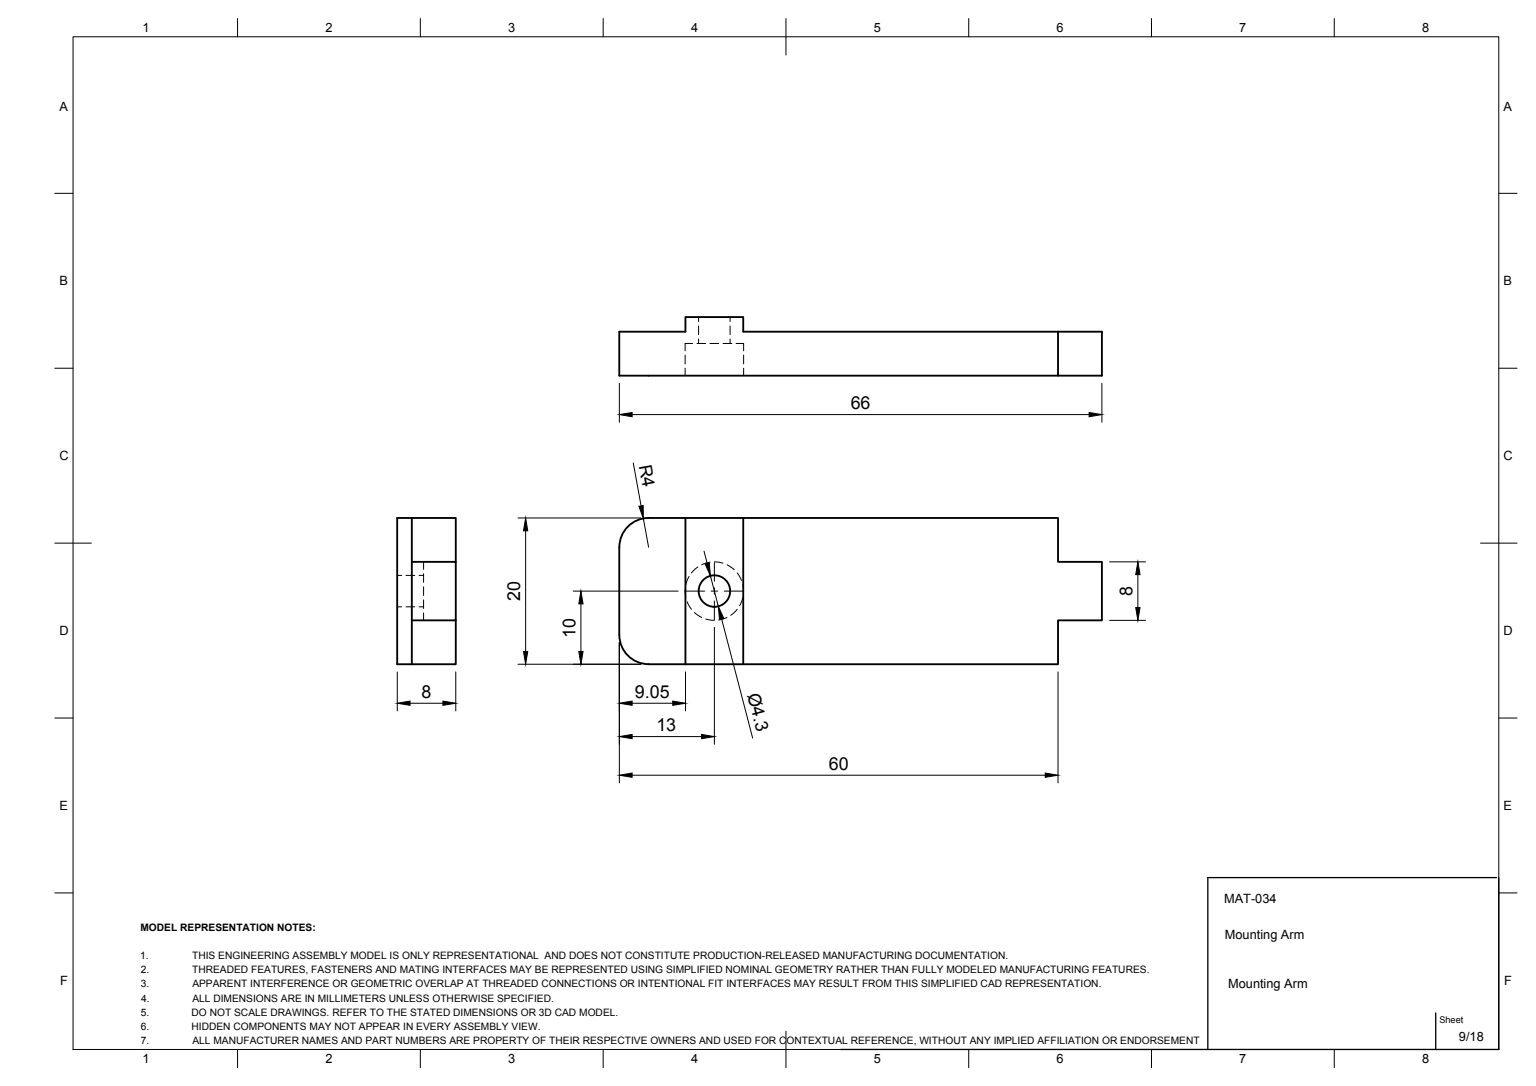
ISO-10303-21;
HEADER;
/* Generated by software containing ST-Developer
 * from STEP Tools, Inc. (www.steptools.com) 
 */

FILE_DESCRIPTION(
/* description */ ('STEP AP214'),
/* implementation_level */ '2;1');

FILE_NAME(
/* name */ 'Mounting Arm.step',
/* time_stamp */ '2026-11-14T09:24:36-08:00',
/* author */ (''),
/* organization */ (''),
/* preprocessor_version */ 'ST-DEVELOPER v20.2',
/* originating_system */ 'Autodesk Translation Framework v15.17.0.0',
/* authorisation */ '');

FILE_SCHEMA (('AUTOMOTIVE_DESIGN { 1 0 10303 214 3 1 1 }'));
ENDSEC;

DATA;
#10=MECHANICAL_DESIGN_GEOMETRIC_PRESENTATION_REPRESENTATION('',(#215),#18867);
#183=SHAPE_REPRESENTATION_RELATIONSHIP('SRR','None',#18947,#199);
#199=ADVANCED_BREP_SHAPE_REPRESENTATION('',(#239),#18863);
#215=STYLED_ITEM('',(#19026),#239);
#239=MANIFOLD_SOLID_BREP('Body1',#10970);
#362=FACE_BOUND('',#1945,.T.);
#363=FACE_BOUND('',#1952,.T.);
#364=FACE_BOUND('',#1956,.T.);
#686=PLANE('',#12091);
#687=PLANE('',#12094);
#688=PLANE('',#12095);
#689=PLANE('',#12096);
#690=PLANE('',#12097);
#691=PLANE('',#12098);
#692=PLANE('',#12099);
#693=PLANE('',#12100);
#694=PLANE('',#12103);
#695=PLANE('',#12104);
#696=PLANE('',#12105);
#697=PLANE('',#12106);
#698=PLANE('',#12107);
#699=PLANE('',#12108);
#700=PLANE('',#12111);
#1228=FACE_OUTER_BOUND('',#1935,.T.);
#1229=FACE_OUTER_BOUND('',#1936,.T.);
#1230=FACE_OUTER_BOUND('',#1937,.T.);
#1231=FACE_OUTER_BOUND('',#1938,.T.);
#1232=FACE_OUTER_BOUND('',#1939,.T.);
#1233=FACE_OUTER_BOUND('',#1940,.T.);
#1234=FACE_OUTER_BOUND('',#1941,.T.);
#1235=FACE_OUTER_BOUND('',#1942,.T.);
#1236=FACE_OUTER_BOUND('',#1943,.T.);
#1237=FACE_OUTER_BOUND('',#1944,.T.);
#1238=FACE_OUTER_BOUND('',#1946,.T.);
#1239=FACE_OUTER_BOUND('',#1947,.T.);
#1240=FACE_OUTER_BOUND('',#1948,.T.);
#1241=FACE_OUTER_BOUND('',#1949,.T.);
#1242=FACE_OUTER_BOUND('',#1950,.T.);
#1243=FACE_OUTER_BOUND('',#1951,.T.);
#1244=FACE_OUTER_BOUND('',#1953,.T.);
#1245=FACE_OUTER_BOUND('',#1954,.T.);
#1246=FACE_OUTER_BOUND('',#1955,.T.);
#1935=EDGE_LOOP('',(#9768,#9769,#9770,#9771));
#1936=EDGE_LOOP('',(#9772,#9773,#9774,#9775));
#1937=EDGE_LOOP('',(#9776,#9777,#9778,#9779,#9780,#9781));
#1938=EDGE_LOOP('',(#9782,#9783,#9784,#9785,#9786,#9787,#9788,#9789));
#1939=EDGE_LOOP('',(#9790,#9791,#9792,#9793));
#1940=EDGE_LOOP('',(#9794,#9795,#9796,#9797));
#1941=EDGE_LOOP('',(#9798,#9799,#9800,#9801,#9802,#9803,#9804,#9805));
#1942=EDGE_LOOP('',(#9806,#9807,#9808,#9809,#9810,#9811,#9812,#9813));
#1943=EDGE_LOOP('',(#9814,#9815,#9816,#9817));
#1944=EDGE_LOOP('',(#9818,#9819,#9820,#9821,#9822,#9823,#9824,#9825,#9826,
#9827));
#1945=EDGE_LOOP('',(#9828));
#1946=EDGE_LOOP('',(#9829,#9830,#9831,#9832));
#1947=EDGE_LOOP('',(#9833,#9834,#9835,#9836));
#1948=EDGE_LOOP('',(#9837,#9838,#9839,#9840));
#1949=EDGE_LOOP('',(#9841,#9842,#9843,#9844));
#1950=EDGE_LOOP('',(#9845,#9846,#9847,#9848));
#1951=EDGE_LOOP('',(#9849,#9850,#9851,#9852));
#1952=EDGE_LOOP('',(#9853));
#1953=EDGE_LOOP('',(#9854,#9855,#9856,#9857));
#1954=EDGE_LOOP('',(#9858,#9859,#9860,#9861));
#1955=EDGE_LOOP('',(#9862));
#1956=EDGE_LOOP('',(#9863));
#2964=LINE('',#18390,#3978);
#2965=LINE('',#18396,#3979);
#2966=LINE('',#18401,#3980);
#2967=LINE('',#18405,#3981);
#2968=LINE('',#18409,#3982);
#2969=LINE('',#18410,#3983);
#2970=LINE('',#18414,#3984);
#2971=LINE('',#18416,#3985);
#2972=LINE('',#18418,#3986);
#2973=LINE('',#18420,#3987);
#2974=LINE('',#18422,#3988);
#2975=LINE('',#18424,#3989);
#2976=LINE('',#18426,#3990);
#2977=LINE('',#18427,#3991);
#2978=LINE('',#18430,#3992);
#2979=LINE('',#18432,#3993);
#2980=LINE('',#18433,#3994);
#2981=LINE('',#18436,#3995);
#2982=LINE('',#18438,#3996);
#2983=LINE('',#18439,#3997);
#2984=LINE('',#18442,#3998);
#2985=LINE('',#18443,#3999);
#2986=LINE('',#18445,#4000);
#2987=LINE('',#18447,#4001);
#2988=LINE('',#18448,#4002);
#2989=LINE('',#18451,#4003);
#2990=LINE('',#18452,#4004);
#2991=LINE('',#18454,#4005);
#2992=LINE('',#18456,#4006);
#2993=LINE('',#18457,#4007);
#2994=LINE('',#18460,#4008);
#2995=LINE('',#18462,#4009);
#2996=LINE('',#18463,#4010);
#2997=LINE('',#18467,#4011);
#2998=LINE('',#18469,#4012);
#2999=LINE('',#18470,#4013);
#3000=LINE('',#18473,#4014);
#3001=LINE('',#18475,#4015);
#3002=LINE('',#18478,#4016);
#3003=LINE('',#18480,#4017);
#3978=VECTOR('',#15076,3.99999999999999);
#3979=VECTOR('',#15083,2.15);
#3980=VECTOR('',#15088,1000.);
#3981=VECTOR('',#15091,1000.);
#3982=VECTOR('',#15094,1000.);
#3983=VECTOR('',#15095,1000.);
#3984=VECTOR('',#15098,1000.);
#3985=VECTOR('',#15099,1000.);
#3986=VECTOR('',#15100,1000.);
#3987=VECTOR('',#15101,1000.);
#3988=VECTOR('',#15102,1000.);
#3989=VECTOR('',#15103,1000.);
#3990=VECTOR('',#15104,1000.);
#3991=VECTOR('',#15105,1000.);
#3992=VECTOR('',#15108,1000.);
#3993=VECTOR('',#15109,1000.);
#3994=VECTOR('',#15110,1000.);
#3995=VECTOR('',#15113,1000.);
#3996=VECTOR('',#15114,1000.);
#3997=VECTOR('',#15115,1000.);
#3998=VECTOR('',#15118,1000.);
#3999=VECTOR('',#15119,1000.);
#4000=VECTOR('',#15120,1000.);
#4001=VECTOR('',#15121,1000.);
#4002=VECTOR('',#15122,1000.);
#4003=VECTOR('',#15125,1000.);
#4004=VECTOR('',#15126,1000.);
#4005=VECTOR('',#15127,1000.);
#4006=VECTOR('',#15128,1000.);
#4007=VECTOR('',#15129,1000.);
#4008=VECTOR('',#15132,1000.);
#4009=VECTOR('',#15133,1000.);
#4010=VECTOR('',#15134,1000.);
#4011=VECTOR('',#15139,1000.);
#4012=VECTOR('',#15140,1000.);
#4013=VECTOR('',#15141,1000.);
#4014=VECTOR('',#15146,1000.);
#4015=VECTOR('',#15149,1000.);
#4016=VECTOR('',#15154,1000.);
#4017=VECTOR('',#15157,1000.);
#4480=CIRCLE('',#12086,4.);
#4481=CIRCLE('',#12087,3.99999999999999);
#4482=CIRCLE('',#12089,2.15);
#4483=CIRCLE('',#12090,2.15);
#4484=CIRCLE('',#12092,4.);
#4485=CIRCLE('',#12093,4.);
#4486=CIRCLE('',#12101,4.);
#4487=CIRCLE('',#12102,4.);
#5456=VERTEX_POINT('',#18387);
#5457=VERTEX_POINT('',#18389);
#5458=VERTEX_POINT('',#18393);
#5459=VERTEX_POINT('',#18395);
#5460=VERTEX_POINT('',#18399);
#5461=VERTEX_POINT('',#18400);
#5462=VERTEX_POINT('',#18402);
#5463=VERTEX_POINT('',#18404);
#5464=VERTEX_POINT('',#18406);
#5465=VERTEX_POINT('',#18408);
#5466=VERTEX_POINT('',#18412);
#5467=VERTEX_POINT('',#18413);
#5468=VERTEX_POINT('',#18415);
#5469=VERTEX_POINT('',#18417);
#5470=VERTEX_POINT('',#18419);
#5471=VERTEX_POINT('',#18421);
#5472=VERTEX_POINT('',#18423);
#5473=VERTEX_POINT('',#18425);
#5474=VERTEX_POINT('',#18429);
#5475=VERTEX_POINT('',#18431);
#5476=VERTEX_POINT('',#18435);
#5477=VERTEX_POINT('',#18437);
#5478=VERTEX_POINT('',#18441);
#5479=VERTEX_POINT('',#18444);
#5480=VERTEX_POINT('',#18446);
#5481=VERTEX_POINT('',#18450);
#5482=VERTEX_POINT('',#18453);
#5483=VERTEX_POINT('',#18455);
#5484=VERTEX_POINT('',#18459);
#5485=VERTEX_POINT('',#18461);
#5486=VERTEX_POINT('',#18466);
#5487=VERTEX_POINT('',#18468);
#6917=EDGE_CURVE('',#5456,#5456,#4480,.T.);
#6918=EDGE_CURVE('',#5456,#5457,#2964,.T.);
#6919=EDGE_CURVE('',#5457,#5457,#4481,.T.);
#6920=EDGE_CURVE('',#5458,#5458,#4482,.T.);
#6921=EDGE_CURVE('',#5458,#5459,#2965,.T.);
#6922=EDGE_CURVE('',#5459,#5459,#4483,.T.);
#6923=EDGE_CURVE('',#5460,#5461,#2966,.T.);
#6924=EDGE_CURVE('',#5460,#5462,#4484,.T.);
#6925=EDGE_CURVE('',#5463,#5462,#2967,.T.);
#6926=EDGE_CURVE('',#5463,#5464,#4485,.T.);
#6927=EDGE_CURVE('',#5465,#5464,#2968,.T.);
#6928=EDGE_CURVE('',#5461,#5465,#2969,.T.);
#6929=EDGE_CURVE('',#5466,#5467,#2970,.T.);
#6930=EDGE_CURVE('',#5468,#5466,#2971,.T.);
#6931=EDGE_CURVE('',#5469,#5468,#2972,.T.);
#6932=EDGE_CURVE('',#5470,#5469,#2973,.T.);
#6933=EDGE_CURVE('',#5471,#5470,#2974,.T.);
#6934=EDGE_CURVE('',#5471,#5472,#2975,.T.);
#6935=EDGE_CURVE('',#5473,#5472,#2976,.T.);
#6936=EDGE_CURVE('',#5467,#5473,#2977,.T.);
#6937=EDGE_CURVE('',#5474,#5472,#2978,.T.);
#6938=EDGE_CURVE('',#5475,#5474,#2979,.T.);
#6939=EDGE_CURVE('',#5475,#5473,#2980,.T.);
#6940=EDGE_CURVE('',#5469,#5476,#2981,.T.);
#6941=EDGE_CURVE('',#5477,#5468,#2982,.T.);
#6942=EDGE_CURVE('',#5476,#5477,#2983,.T.);
#6943=EDGE_CURVE('',#5478,#5475,#2984,.T.);
#6944=EDGE_CURVE('',#5478,#5460,#2985,.T.);
#6945=EDGE_CURVE('',#5479,#5461,#2986,.T.);
#6946=EDGE_CURVE('',#5480,#5479,#2987,.T.);
#6947=EDGE_CURVE('',#5480,#5467,#2988,.T.);
#6948=EDGE_CURVE('',#5464,#5481,#2989,.T.);
#6949=EDGE_CURVE('',#5477,#5481,#2990,.T.);
#6950=EDGE_CURVE('',#5482,#5466,#2991,.T.);
#6951=EDGE_CURVE('',#5483,#5482,#2992,.T.);
#6952=EDGE_CURVE('',#5483,#5465,#2993,.T.);
#6953=EDGE_CURVE('',#5462,#5484,#2994,.T.);
#6954=EDGE_CURVE('',#5485,#5484,#2995,.T.);
#6955=EDGE_CURVE('',#5485,#5463,#2996,.T.);
#6956=EDGE_CURVE('',#5484,#5478,#4486,.T.);
#6957=EDGE_CURVE('',#5486,#5474,#2997,.T.);
#6958=EDGE_CURVE('',#5487,#5486,#2998,.T.);
#6959=EDGE_CURVE('',#5487,#5476,#2999,.T.);
#6960=EDGE_CURVE('',#5481,#5485,#4487,.T.);
#6961=EDGE_CURVE('',#5486,#5471,#3000,.T.);
#6962=EDGE_CURVE('',#5470,#5487,#3001,.T.);
#6963=EDGE_CURVE('',#5482,#5480,#3002,.T.);
#6964=EDGE_CURVE('',#5479,#5483,#3003,.T.);
#9768=ORIENTED_EDGE('',*,*,#6917,.F.);
#9769=ORIENTED_EDGE('',*,*,#6918,.T.);
#9770=ORIENTED_EDGE('',*,*,#6919,.T.);
#9771=ORIENTED_EDGE('',*,*,#6918,.F.);
#9772=ORIENTED_EDGE('',*,*,#6920,.F.);
#9773=ORIENTED_EDGE('',*,*,#6921,.T.);
#9774=ORIENTED_EDGE('',*,*,#6922,.T.);
#9775=ORIENTED_EDGE('',*,*,#6921,.F.);
#9776=ORIENTED_EDGE('',*,*,#6923,.F.);
#9777=ORIENTED_EDGE('',*,*,#6924,.T.);
#9778=ORIENTED_EDGE('',*,*,#6925,.F.);
#9779=ORIENTED_EDGE('',*,*,#6926,.T.);
#9780=ORIENTED_EDGE('',*,*,#6927,.F.);
#9781=ORIENTED_EDGE('',*,*,#6928,.F.);
#9782=ORIENTED_EDGE('',*,*,#6929,.F.);
#9783=ORIENTED_EDGE('',*,*,#6930,.F.);
#9784=ORIENTED_EDGE('',*,*,#6931,.F.);
#9785=ORIENTED_EDGE('',*,*,#6932,.F.);
#9786=ORIENTED_EDGE('',*,*,#6933,.F.);
#9787=ORIENTED_EDGE('',*,*,#6934,.T.);
#9788=ORIENTED_EDGE('',*,*,#6935,.F.);
#9789=ORIENTED_EDGE('',*,*,#6936,.F.);
#9790=ORIENTED_EDGE('',*,*,#6937,.F.);
#9791=ORIENTED_EDGE('',*,*,#6938,.F.);
#9792=ORIENTED_EDGE('',*,*,#6939,.T.);
#9793=ORIENTED_EDGE('',*,*,#6935,.T.);
#9794=ORIENTED_EDGE('',*,*,#6940,.F.);
#9795=ORIENTED_EDGE('',*,*,#6931,.T.);
#9796=ORIENTED_EDGE('',*,*,#6941,.F.);
#9797=ORIENTED_EDGE('',*,*,#6942,.F.);
#9798=ORIENTED_EDGE('',*,*,#6943,.F.);
#9799=ORIENTED_EDGE('',*,*,#6944,.T.);
#9800=ORIENTED_EDGE('',*,*,#6923,.T.);
#9801=ORIENTED_EDGE('',*,*,#6945,.F.);
#9802=ORIENTED_EDGE('',*,*,#6946,.F.);
#9803=ORIENTED_EDGE('',*,*,#6947,.T.);
#9804=ORIENTED_EDGE('',*,*,#6936,.T.);
#9805=ORIENTED_EDGE('',*,*,#6939,.F.);
#9806=ORIENTED_EDGE('',*,*,#6927,.T.);
#9807=ORIENTED_EDGE('',*,*,#6948,.T.);
#9808=ORIENTED_EDGE('',*,*,#6949,.F.);
#9809=ORIENTED_EDGE('',*,*,#6941,.T.);
#9810=ORIENTED_EDGE('',*,*,#6930,.T.);
#9811=ORIENTED_EDGE('',*,*,#6950,.F.);
#9812=ORIENTED_EDGE('',*,*,#6951,.F.);
#9813=ORIENTED_EDGE('',*,*,#6952,.T.);
#9814=ORIENTED_EDGE('',*,*,#6925,.T.);
#9815=ORIENTED_EDGE('',*,*,#6953,.T.);
#9816=ORIENTED_EDGE('',*,*,#6954,.F.);
#9817=ORIENTED_EDGE('',*,*,#6955,.T.);
#9818=ORIENTED_EDGE('',*,*,#6954,.T.);
#9819=ORIENTED_EDGE('',*,*,#6956,.T.);
#9820=ORIENTED_EDGE('',*,*,#6943,.T.);
#9821=ORIENTED_EDGE('',*,*,#6938,.T.);
#9822=ORIENTED_EDGE('',*,*,#6957,.F.);
#9823=ORIENTED_EDGE('',*,*,#6958,.F.);
#9824=ORIENTED_EDGE('',*,*,#6959,.T.);
#9825=ORIENTED_EDGE('',*,*,#6942,.T.);
#9826=ORIENTED_EDGE('',*,*,#6949,.T.);
#9827=ORIENTED_EDGE('',*,*,#6960,.T.);
#9828=ORIENTED_EDGE('',*,*,#6919,.F.);
#9829=ORIENTED_EDGE('',*,*,#6937,.T.);
#9830=ORIENTED_EDGE('',*,*,#6934,.F.);
#9831=ORIENTED_EDGE('',*,*,#6961,.F.);
#9832=ORIENTED_EDGE('',*,*,#6957,.T.);
#9833=ORIENTED_EDGE('',*,*,#6940,.T.);
#9834=ORIENTED_EDGE('',*,*,#6959,.F.);
#9835=ORIENTED_EDGE('',*,*,#6962,.F.);
#9836=ORIENTED_EDGE('',*,*,#6932,.T.);
#9837=ORIENTED_EDGE('',*,*,#6961,.T.);
#9838=ORIENTED_EDGE('',*,*,#6933,.T.);
#9839=ORIENTED_EDGE('',*,*,#6962,.T.);
#9840=ORIENTED_EDGE('',*,*,#6958,.T.);
#9841=ORIENTED_EDGE('',*,*,#6929,.T.);
#9842=ORIENTED_EDGE('',*,*,#6947,.F.);
#9843=ORIENTED_EDGE('',*,*,#6963,.F.);
#9844=ORIENTED_EDGE('',*,*,#6950,.T.);
#9845=ORIENTED_EDGE('',*,*,#6928,.T.);
#9846=ORIENTED_EDGE('',*,*,#6952,.F.);
#9847=ORIENTED_EDGE('',*,*,#6964,.F.);
#9848=ORIENTED_EDGE('',*,*,#6945,.T.);
#9849=ORIENTED_EDGE('',*,*,#6951,.T.);
#9850=ORIENTED_EDGE('',*,*,#6963,.T.);
#9851=ORIENTED_EDGE('',*,*,#6946,.T.);
#9852=ORIENTED_EDGE('',*,*,#6964,.T.);
#9853=ORIENTED_EDGE('',*,*,#6920,.T.);
#9854=ORIENTED_EDGE('',*,*,#6956,.F.);
#9855=ORIENTED_EDGE('',*,*,#6953,.F.);
#9856=ORIENTED_EDGE('',*,*,#6924,.F.);
#9857=ORIENTED_EDGE('',*,*,#6944,.F.);
#9858=ORIENTED_EDGE('',*,*,#6960,.F.);
#9859=ORIENTED_EDGE('',*,*,#6948,.F.);
#9860=ORIENTED_EDGE('',*,*,#6926,.F.);
#9861=ORIENTED_EDGE('',*,*,#6955,.F.);
#9862=ORIENTED_EDGE('',*,*,#6917,.T.);
#9863=ORIENTED_EDGE('',*,*,#6922,.F.);
#10337=CYLINDRICAL_SURFACE('',#12085,3.99999999999999);
#10338=CYLINDRICAL_SURFACE('',#12088,2.15);
#10339=CYLINDRICAL_SURFACE('',#12109,4.);
#10340=CYLINDRICAL_SURFACE('',#12110,4.);
#10865=ADVANCED_FACE('',(#1228),#10337,.F.);
#10866=ADVANCED_FACE('',(#1229),#10338,.F.);
#10867=ADVANCED_FACE('',(#1230),#686,.F.);
#10868=ADVANCED_FACE('',(#1231),#687,.F.);
#10869=ADVANCED_FACE('',(#1232),#688,.F.);
#10870=ADVANCED_FACE('',(#1233),#689,.F.);
#10871=ADVANCED_FACE('',(#1234),#690,.F.);
#10872=ADVANCED_FACE('',(#1235),#691,.F.);
#10873=ADVANCED_FACE('',(#1236),#692,.F.);
#10874=ADVANCED_FACE('',(#1237,#362),#693,.T.);
#10875=ADVANCED_FACE('',(#1238),#694,.F.);
#10876=ADVANCED_FACE('',(#1239),#695,.F.);
#10877=ADVANCED_FACE('',(#1240),#696,.T.);
#10878=ADVANCED_FACE('',(#1241),#697,.F.);
#10879=ADVANCED_FACE('',(#1242),#698,.F.);
#10880=ADVANCED_FACE('',(#1243,#363),#699,.T.);
#10881=ADVANCED_FACE('',(#1244),#10339,.T.);
#10882=ADVANCED_FACE('',(#1245),#10340,.T.);
#10883=ADVANCED_FACE('',(#1246,#364),#700,.F.);
#10970=CLOSED_SHELL('',(#10865,#10866,#10867,#10868,#10869,#10870,#10871,
#10872,#10873,#10874,#10875,#10876,#10877,#10878,#10879,#10880,#10881,#10882,
#10883));
#12084=AXIS2_PLACEMENT_3D('',#18385,#15070,#15071);
#12085=AXIS2_PLACEMENT_3D('',#18386,#15072,#15073);
#12086=AXIS2_PLACEMENT_3D('',#18388,#15074,#15075);
#12087=AXIS2_PLACEMENT_3D('',#18391,#15077,#15078);
#12088=AXIS2_PLACEMENT_3D('',#18392,#15079,#15080);
#12089=AXIS2_PLACEMENT_3D('',#18394,#15081,#15082);
#12090=AXIS2_PLACEMENT_3D('',#18397,#15084,#15085);
#12091=AXIS2_PLACEMENT_3D('',#18398,#15086,#15087);
#12092=AXIS2_PLACEMENT_3D('',#18403,#15089,#15090);
#12093=AXIS2_PLACEMENT_3D('',#18407,#15092,#15093);
#12094=AXIS2_PLACEMENT_3D('',#18411,#15096,#15097);
#12095=AXIS2_PLACEMENT_3D('',#18428,#15106,#15107);
#12096=AXIS2_PLACEMENT_3D('',#18434,#15111,#15112);
#12097=AXIS2_PLACEMENT_3D('',#18440,#15116,#15117);
#12098=AXIS2_PLACEMENT_3D('',#18449,#15123,#15124);
#12099=AXIS2_PLACEMENT_3D('',#18458,#15130,#15131);
#12100=AXIS2_PLACEMENT_3D('',#18464,#15135,#15136);
#12101=AXIS2_PLACEMENT_3D('',#18465,#15137,#15138);
#12102=AXIS2_PLACEMENT_3D('',#18471,#15142,#15143);
#12103=AXIS2_PLACEMENT_3D('',#18472,#15144,#15145);
#12104=AXIS2_PLACEMENT_3D('',#18474,#15147,#15148);
#12105=AXIS2_PLACEMENT_3D('',#18476,#15150,#15151);
#12106=AXIS2_PLACEMENT_3D('',#18477,#15152,#15153);
#12107=AXIS2_PLACEMENT_3D('',#18479,#15155,#15156);
#12108=AXIS2_PLACEMENT_3D('',#18481,#15158,#15159);
#12109=AXIS2_PLACEMENT_3D('',#18482,#15160,#15161);
#12110=AXIS2_PLACEMENT_3D('',#18483,#15162,#15163);
#12111=AXIS2_PLACEMENT_3D('',#18484,#15164,#15165);
#15070=DIRECTION('axis',(0.,0.,1.));
#15071=DIRECTION('refdir',(1.,0.,0.));
#15072=DIRECTION('center_axis',(0.,0.,1.));
#15073=DIRECTION('ref_axis',(1.,0.,0.));
#15074=DIRECTION('center_axis',(0.,0.,1.));
#15075=DIRECTION('ref_axis',(1.,0.,0.));
#15076=DIRECTION('',(0.,0.,1.));
#15077=DIRECTION('center_axis',(0.,0.,1.));
#15078=DIRECTION('ref_axis',(1.,0.,0.));
#15079=DIRECTION('center_axis',(0.,0.,1.));
#15080=DIRECTION('ref_axis',(1.,0.,0.));
#15081=DIRECTION('center_axis',(0.,0.,1.));
#15082=DIRECTION('ref_axis',(1.,0.,0.));
#15083=DIRECTION('',(0.,0.,1.));
#15084=DIRECTION('center_axis',(0.,0.,1.));
#15085=DIRECTION('ref_axis',(1.,0.,0.));
#15086=DIRECTION('center_axis',(0.,0.,1.));
#15087=DIRECTION('ref_axis',(1.,0.,0.));
#15088=DIRECTION('',(0.,-1.,0.));
#15089=DIRECTION('center_axis',(0.,0.,-1.));
#15090=DIRECTION('ref_axis',(1.,0.,0.));
#15091=DIRECTION('',(-1.,0.,0.));
#15092=DIRECTION('center_axis',(0.,0.,-1.));
#15093=DIRECTION('ref_axis',(1.,2.60208521396521E-15,0.));
#15094=DIRECTION('',(0.,1.,0.));
#15095=DIRECTION('',(1.,-1.73472347597681E-16,0.));
#15096=DIRECTION('center_axis',(0.,0.,1.));
#15097=DIRECTION('ref_axis',(1.,0.,0.));
#15098=DIRECTION('',(-1.,0.,0.));
#15099=DIRECTION('',(0.,1.,0.));
#15100=DIRECTION('',(1.,1.73472347597681E-16,0.));
#15101=DIRECTION('',(-8.67361737988404E-17,1.,0.));
#15102=DIRECTION('',(1.,0.,1.26217744835362E-26));
#15103=DIRECTION('',(-8.67361737988404E-17,1.,0.));
#15104=DIRECTION('',(1.,1.73472347597681E-16,0.));
#15105=DIRECTION('',(0.,-1.,0.));
#15106=DIRECTION('center_axis',(-1.73472347597681E-16,1.,0.));
#15107=DIRECTION('ref_axis',(-1.,-1.73472347597681E-16,0.));
#15108=DIRECTION('',(0.,0.,-1.));
#15109=DIRECTION('',(1.,1.73472347597681E-16,0.));
#15110=DIRECTION('',(0.,0.,-1.));
#15111=DIRECTION('center_axis',(-1.73472347597681E-16,1.,0.));
#15112=DIRECTION('ref_axis',(-1.,-1.73472347597681E-16,0.));
#15113=DIRECTION('',(0.,0.,1.));
#15114=DIRECTION('',(0.,0.,-1.));
#15115=DIRECTION('',(1.,1.73472347597681E-16,0.));
#15116=DIRECTION('center_axis',(1.,0.,0.));
#15117=DIRECTION('ref_axis',(0.,0.,-1.));
#15118=DIRECTION('',(0.,-1.,0.));
#15119=DIRECTION('',(0.,0.,-1.));
#15120=DIRECTION('',(0.,0.,1.));
#15121=DIRECTION('',(0.,1.,0.));
#15122=DIRECTION('',(0.,0.,1.));
#15123=DIRECTION('center_axis',(-1.,0.,0.));
#15124=DIRECTION('ref_axis',(0.,0.,1.));
#15125=DIRECTION('',(0.,0.,1.));
#15126=DIRECTION('',(0.,1.,0.));
#15127=DIRECTION('',(0.,0.,1.));
#15128=DIRECTION('',(-2.19585250123647E-16,-1.,0.));
#15129=DIRECTION('',(0.,0.,1.));
#15130=DIRECTION('center_axis',(0.,-1.,0.));
#15131=DIRECTION('ref_axis',(0.,0.,-1.));
#15132=DIRECTION('',(0.,0.,1.));
#15133=DIRECTION('',(-1.,0.,0.));
#15134=DIRECTION('',(0.,0.,-1.));
#15135=DIRECTION('center_axis',(0.,0.,1.));
#15136=DIRECTION('ref_axis',(1.,0.,0.));
#15137=DIRECTION('center_axis',(0.,0.,1.));
#15138=DIRECTION('ref_axis',(1.,0.,0.));
#15139=DIRECTION('',(-8.67361737988404E-17,1.,0.));
#15140=DIRECTION('',(-1.,0.,0.));
#15141=DIRECTION('',(-8.67361737988404E-17,1.,0.));
#15142=DIRECTION('center_axis',(0.,0.,1.));
#15143=DIRECTION('ref_axis',(1.,0.,0.));
#15144=DIRECTION('center_axis',(1.,8.67361737988403E-17,0.));
#15145=DIRECTION('ref_axis',(-8.67361737988404E-17,1.,0.));
#15146=DIRECTION('',(0.,0.,-1.));
#15147=DIRECTION('center_axis',(-1.,-8.67361737988403E-17,0.));
#15148=DIRECTION('ref_axis',(8.67361737988404E-17,-1.,0.));
#15149=DIRECTION('',(0.,0.,1.));
#15150=DIRECTION('center_axis',(0.,-1.,0.));
#15151=DIRECTION('ref_axis',(0.,0.,-1.));
#15152=DIRECTION('center_axis',(0.,1.,0.));
#15153=DIRECTION('ref_axis',(0.,0.,1.));
#15154=DIRECTION('',(-1.,0.,0.));
#15155=DIRECTION('center_axis',(-1.73472347597681E-16,-1.,0.));
#15156=DIRECTION('ref_axis',(1.,-1.73472347597681E-16,0.));
#15157=DIRECTION('',(1.,-1.73472347597681E-16,0.));
#15158=DIRECTION('center_axis',(0.,0.,-1.));
#15159=DIRECTION('ref_axis',(-1.,0.,0.));
#15160=DIRECTION('center_axis',(0.,0.,-1.));
#15161=DIRECTION('ref_axis',(-1.,0.,0.));
#15162=DIRECTION('center_axis',(0.,0.,-1.));
#15163=DIRECTION('ref_axis',(-1.,0.,0.));
#15164=DIRECTION('center_axis',(0.,0.,-1.));
#15165=DIRECTION('ref_axis',(-1.,0.,0.));
#18385=CARTESIAN_POINT('',(0.,0.,0.));
#18386=CARTESIAN_POINT('Origin',(0.,17.,6.));
#18387=CARTESIAN_POINT('',(-3.99999999999999,17.,1.6));
#18388=CARTESIAN_POINT('Origin',(0.,17.,1.6));
#18389=CARTESIAN_POINT('',(-3.99999999999999,17.,6.));
#18390=CARTESIAN_POINT('',(-3.99999999999999,17.,6.));
#18391=CARTESIAN_POINT('Origin',(0.,17.,6.));
#18392=CARTESIAN_POINT('Origin',(0.,17.,6.));
#18393=CARTESIAN_POINT('',(-2.15,17.,-2.));
#18394=CARTESIAN_POINT('Origin',(0.,17.,-2.));
#18395=CARTESIAN_POINT('',(-2.15,17.,1.6));
#18396=CARTESIAN_POINT('',(-2.15,17.,6.));
#18397=CARTESIAN_POINT('Origin',(0.,17.,1.6));
#18398=CARTESIAN_POINT('Origin',(0.,0.,0.));
#18399=CARTESIAN_POINT('',(-10.,26.,0.));
#18400=CARTESIAN_POINT('',(-10.,20.95,0.));
#18401=CARTESIAN_POINT('',(-10.,-30.,0.));
#18402=CARTESIAN_POINT('',(-6.,30.,0.));
#18403=CARTESIAN_POINT('Origin',(-6.,26.,0.));
#18404=CARTESIAN_POINT('',(6.,30.,0.));
#18405=CARTESIAN_POINT('',(10.,30.,0.));
#18406=CARTESIAN_POINT('',(10.,26.,0.));
#18407=CARTESIAN_POINT('Origin',(6.,26.,0.));
#18408=CARTESIAN_POINT('',(10.,20.95,0.));
#18409=CARTESIAN_POINT('',(10.,-30.,0.));
#18410=CARTESIAN_POINT('',(10.,20.95,0.));
#18411=CARTESIAN_POINT('Origin',(0.,0.,0.));
#18412=CARTESIAN_POINT('',(10.,13.05,0.));
#18413=CARTESIAN_POINT('',(-10.,13.05,0.));
#18414=CARTESIAN_POINT('',(10.,13.05,0.));
#18415=CARTESIAN_POINT('',(10.,-30.,0.));
#18416=CARTESIAN_POINT('',(10.,-30.,0.));
#18417=CARTESIAN_POINT('',(4.00000000000001,-30.,0.));
#18418=CARTESIAN_POINT('',(10.,-30.,0.));
#18419=CARTESIAN_POINT('',(4.00000000000001,-36.,4.54060943916541E-16));
#18420=CARTESIAN_POINT('',(4.00000000000001,-36.,4.54060943916541E-16));
#18421=CARTESIAN_POINT('',(-3.99999999999999,-36.,4.54060943815567E-16));
#18422=CARTESIAN_POINT('',(4.00000000000001,-36.,4.54060943916541E-16));
#18423=CARTESIAN_POINT('',(-3.99999999999999,-30.,0.));
#18424=CARTESIAN_POINT('',(-3.99999999999999,-36.,4.54060943815567E-16));
#18425=CARTESIAN_POINT('',(-10.,-30.,0.));
#18426=CARTESIAN_POINT('',(10.,-30.,0.));
#18427=CARTESIAN_POINT('',(-10.,-30.,0.));
#18428=CARTESIAN_POINT('Origin',(10.,-30.,6.));
#18429=CARTESIAN_POINT('',(-3.99999999999999,-30.,6.));
#18430=CARTESIAN_POINT('',(-3.99999999999999,-30.,4.54060943815567E-16));
#18431=CARTESIAN_POINT('',(-10.,-30.,6.));
#18432=CARTESIAN_POINT('',(10.,-30.,6.));
#18433=CARTESIAN_POINT('',(-10.,-30.,6.));
#18434=CARTESIAN_POINT('Origin',(10.,-30.,6.));
#18435=CARTESIAN_POINT('',(4.00000000000001,-30.,6.));
#18436=CARTESIAN_POINT('',(4.00000000000001,-30.,4.54060943916541E-16));
#18437=CARTESIAN_POINT('',(10.,-30.,6.));
#18438=CARTESIAN_POINT('',(10.,-30.,6.));
#18439=CARTESIAN_POINT('',(10.,-30.,6.));
#18440=CARTESIAN_POINT('Origin',(-10.,-30.,6.));
#18441=CARTESIAN_POINT('',(-10.,26.,6.));
#18442=CARTESIAN_POINT('',(-10.,-30.,6.));
#18443=CARTESIAN_POINT('',(-10.,26.,6.));
#18444=CARTESIAN_POINT('',(-10.,20.95,-2.));
#18445=CARTESIAN_POINT('',(-10.,20.95,-2.));
#18446=CARTESIAN_POINT('',(-10.,13.05,-2.));
#18447=CARTESIAN_POINT('',(-10.,20.95,-2.));
#18448=CARTESIAN_POINT('',(-10.,13.05,-2.));
#18449=CARTESIAN_POINT('Origin',(10.,-30.,6.));
#18450=CARTESIAN_POINT('',(10.,26.,6.));
#18451=CARTESIAN_POINT('',(10.,26.,6.));
#18452=CARTESIAN_POINT('',(10.,-30.,6.));
#18453=CARTESIAN_POINT('',(10.,13.05,-2.));
#18454=CARTESIAN_POINT('',(10.,13.05,-2.));
#18455=CARTESIAN_POINT('',(10.,20.95,-2.));
#18456=CARTESIAN_POINT('',(10.,20.95,-2.));
#18457=CARTESIAN_POINT('',(10.,20.95,-2.));
#18458=CARTESIAN_POINT('Origin',(10.,30.,6.));
#18459=CARTESIAN_POINT('',(-6.,30.,6.));
#18460=CARTESIAN_POINT('',(-6.,30.,6.));
#18461=CARTESIAN_POINT('',(6.,30.,6.));
#18462=CARTESIAN_POINT('',(10.,30.,6.));
#18463=CARTESIAN_POINT('',(6.,30.,6.));
#18464=CARTESIAN_POINT('Origin',(0.,0.,6.));
#18465=CARTESIAN_POINT('Origin',(-6.,26.,6.));
#18466=CARTESIAN_POINT('',(-3.99999999999999,-36.,6.));
#18467=CARTESIAN_POINT('',(-3.99999999999999,-36.,6.));
#18468=CARTESIAN_POINT('',(4.00000000000001,-36.,6.));
#18469=CARTESIAN_POINT('',(4.00000000000001,-36.,6.));
#18470=CARTESIAN_POINT('',(4.00000000000001,-36.,6.));
#18471=CARTESIAN_POINT('Origin',(6.,26.,6.));
#18472=CARTESIAN_POINT('Origin',(-3.99999999999999,-36.,4.54060943815567E-16));
#18473=CARTESIAN_POINT('',(-3.99999999999999,-36.,4.54060943815567E-16));
#18474=CARTESIAN_POINT('Origin',(4.00000000000001,-36.,4.54060943916541E-16));
#18475=CARTESIAN_POINT('',(4.00000000000001,-36.,4.54060943916541E-16));
#18476=CARTESIAN_POINT('Origin',(5.20417042793042E-16,-36.,0.));
#18477=CARTESIAN_POINT('Origin',(10.,13.05,-2.));
#18478=CARTESIAN_POINT('',(10.,13.05,-2.));
#18479=CARTESIAN_POINT('Origin',(10.,20.95,-2.));
#18480=CARTESIAN_POINT('',(10.,20.95,-2.));
#18481=CARTESIAN_POINT('Origin',(0.,0.,-2.));
#18482=CARTESIAN_POINT('Origin',(-6.,26.,6.));
#18483=CARTESIAN_POINT('Origin',(6.,26.,6.));
#18484=CARTESIAN_POINT('Origin',(2.15,17.,1.6));
#18845=UNCERTAINTY_MEASURE_WITH_UNIT(LENGTH_MEASURE(0.01),#18868,
'DISTANCE_ACCURACY_VALUE',
'Maximum model space distance between geometric entities at asserted c
onnectivities');
#18849=UNCERTAINTY_MEASURE_WITH_UNIT(LENGTH_MEASURE(0.01),#18868,
'DISTANCE_ACCURACY_VALUE',
'Maximum model space distance between geometric entities at asserted c
onnectivities');
#18863=(
GEOMETRIC_REPRESENTATION_CONTEXT(3)
GLOBAL_UNCERTAINTY_ASSIGNED_CONTEXT((#18845))
GLOBAL_UNIT_ASSIGNED_CONTEXT((#18868,#18870,#18871))
REPRESENTATION_CONTEXT('','3D')
);
#18867=(
GEOMETRIC_REPRESENTATION_CONTEXT(3)
GLOBAL_UNCERTAINTY_ASSIGNED_CONTEXT((#18849))
GLOBAL_UNIT_ASSIGNED_CONTEXT((#18868,#18870,#18871))
REPRESENTATION_CONTEXT('','3D')
);
#18868=(
LENGTH_UNIT()
NAMED_UNIT(*)
SI_UNIT(.MILLI.,.METRE.)
);
#18870=(
NAMED_UNIT(*)
PLANE_ANGLE_UNIT()
SI_UNIT($,.RADIAN.)
);
#18871=(
NAMED_UNIT(*)
SI_UNIT($,.STERADIAN.)
SOLID_ANGLE_UNIT()
);
#18885=SHAPE_DEFINITION_REPRESENTATION(#18902,#18947);
#18902=PRODUCT_DEFINITION_SHAPE('',$,#18965);
#18947=SHAPE_REPRESENTATION('',(#12084),#18863);
#18951=PRODUCT_DEFINITION_CONTEXT('part definition',#19004,'design');
#18965=PRODUCT_DEFINITION('Mounting Arm','Mounting Arm',#18982,#18951);
#18982=PRODUCT_DEFINITION_FORMATION('',$,#19019);
#19004=APPLICATION_CONTEXT(
'Core Data for Automotive Mechanical Design Process');
#19005=PRODUCT_CONTEXT('part definition',#19004,'mechanical');
#19019=PRODUCT('Mounting Arm','Mounting Arm',$,(#19005));
#19026=PRESENTATION_STYLE_ASSIGNMENT((#19032));
#19032=SURFACE_STYLE_USAGE(.BOTH.,#19038);
#19038=SURFACE_SIDE_STYLE('',(#19044));
#19044=SURFACE_STYLE_FILL_AREA(#19050);
#19050=FILL_AREA_STYLE('Opaque(227,224,212)',(#19056));
#19056=FILL_AREA_STYLE_COLOUR('Opaque(227,224,212)',#19062);
#19062=COLOUR_RGB('Opaque(227,224,212)',0.890196078431372,0.87843137254902,
0.831372549019608);
ENDSEC;
END-ISO-10303-21;
